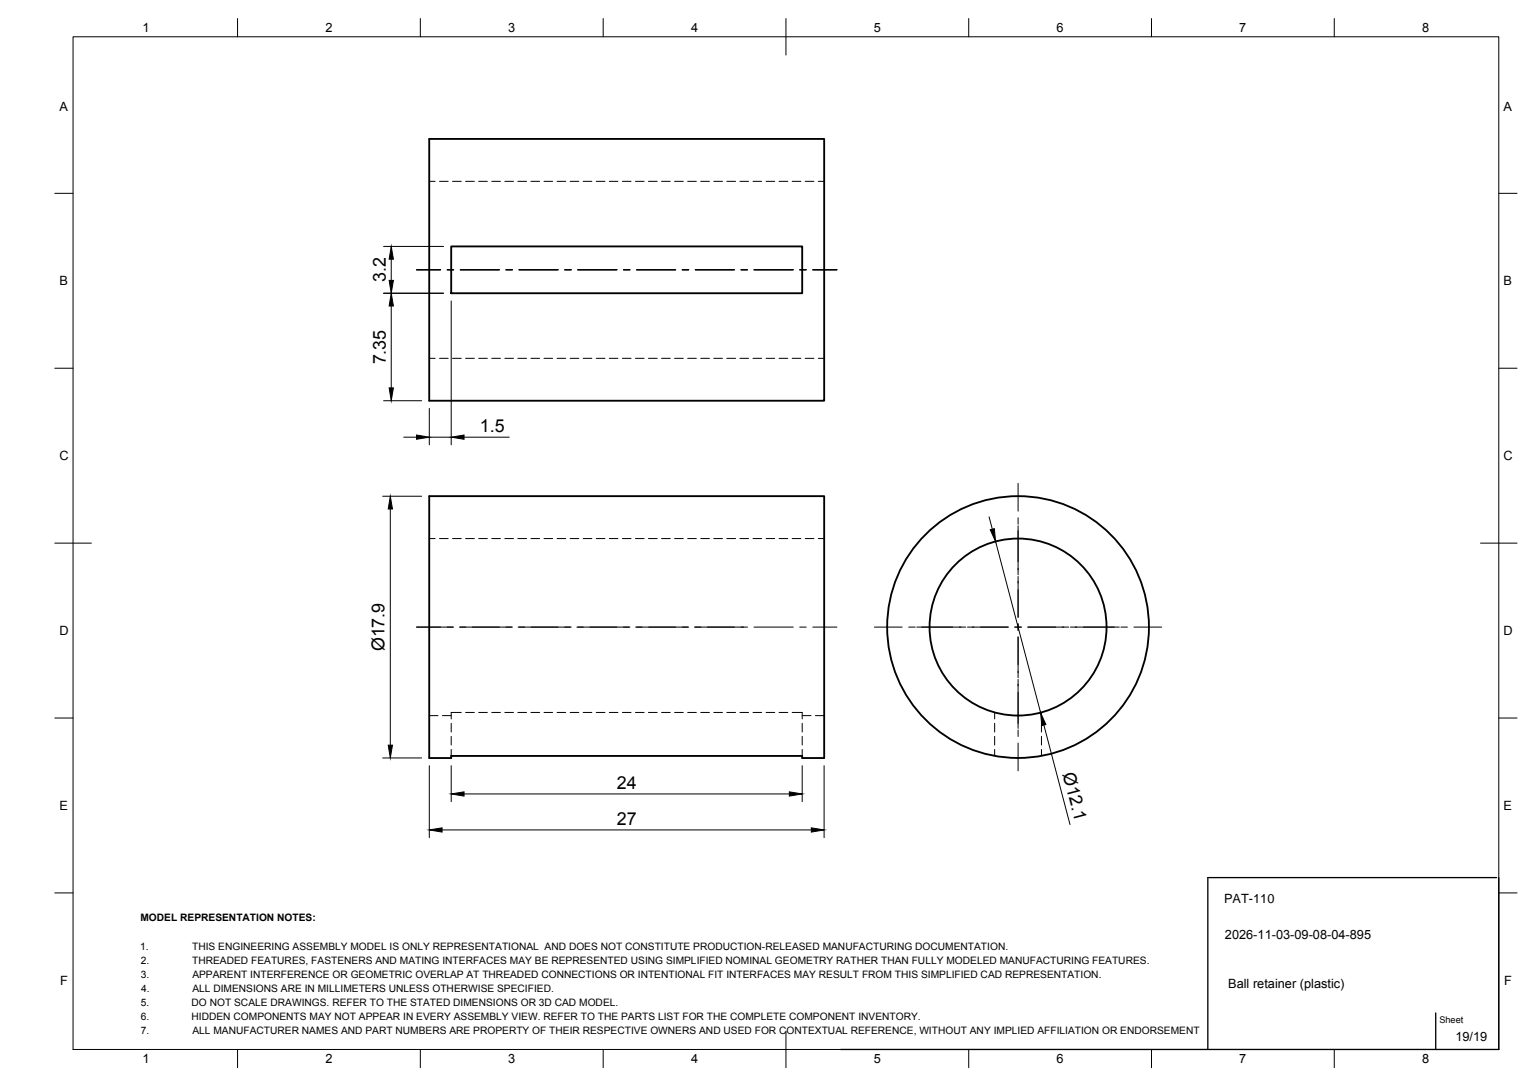
ISO-10303-21;
HEADER;
/* Generated by software containing ST-Developer
 * from STEP Tools, Inc. (www.steptools.com) 
 */

FILE_DESCRIPTION(
/* description */ ('Twin-shaft manual slide'),
/* implementation_level */ '2;1');

FILE_NAME(
/* name */ 'Ball retainer (plastic).step',
/* time_stamp */ '2026-10-27T18:38:08-07:00',
/* author */ (''),
/* organization */ (''),
/* preprocessor_version */ 'ST-DEVELOPER v20.2',
/* originating_system */ 'Autodesk Translation Framework v15.17.0.0',
/* authorisation */ '');

FILE_SCHEMA (('AUTOMOTIVE_DESIGN { 1 0 10303 214 3 1 1 }'));
ENDSEC;

DATA;
#10=MECHANICAL_DESIGN_GEOMETRIC_PRESENTATION_REPRESENTATION('',(#285),#6463);
#253=SHAPE_REPRESENTATION_RELATIONSHIP('SRR','None',#6573,#269);
#269=ADVANCED_BREP_SHAPE_REPRESENTATION('',(#300),#6456);
#285=STYLED_ITEM('',(#6733),#300);
#300=MANIFOLD_SOLID_BREP('Body1',#3648);
#378=FACE_BOUND('',#940,.T.);
#379=FACE_BOUND('',#942,.T.);
#380=FACE_BOUND('',#944,.T.);
#381=FACE_BOUND('',#946,.T.);
#477=PLANE('',#4078);
#478=PLANE('',#4081);
#479=PLANE('',#4082);
#480=PLANE('',#4085);
#481=PLANE('',#4086);
#482=PLANE('',#4091);
#654=FACE_OUTER_BOUND('',#935,.T.);
#655=FACE_OUTER_BOUND('',#936,.T.);
#656=FACE_OUTER_BOUND('',#937,.T.);
#657=FACE_OUTER_BOUND('',#938,.T.);
#658=FACE_OUTER_BOUND('',#939,.T.);
#659=FACE_OUTER_BOUND('',#941,.T.);
#660=FACE_OUTER_BOUND('',#943,.T.);
#661=FACE_OUTER_BOUND('',#945,.T.);
#935=EDGE_LOOP('',(#3054,#3055,#3056,#3057));
#936=EDGE_LOOP('',(#3058,#3059,#3060,#3061));
#937=EDGE_LOOP('',(#3062,#3063,#3064,#3065));
#938=EDGE_LOOP('',(#3066,#3067,#3068,#3069));
#939=EDGE_LOOP('',(#3070));
#940=EDGE_LOOP('',(#3071));
#941=EDGE_LOOP('',(#3072,#3073,#3074,#3075));
#942=EDGE_LOOP('',(#3076,#3077,#3078,#3079));
#943=EDGE_LOOP('',(#3080));
#944=EDGE_LOOP('',(#3081));
#945=EDGE_LOOP('',(#3082,#3083,#3084,#3085));
#946=EDGE_LOOP('',(#3086,#3087,#3088,#3089));
#1219=LINE('',#6034,#1505);
#1220=LINE('',#6037,#1506);
#1221=LINE('',#6040,#1507);
#1222=LINE('',#6042,#1508);
#1223=LINE('',#6043,#1509);
#1224=LINE('',#6049,#1510);
#1225=LINE('',#6051,#1511);
#1226=LINE('',#6052,#1512);
#1227=LINE('',#6061,#1513);
#1228=LINE('',#6066,#1514);
#1505=VECTOR('',#4939,1.);
#1506=VECTOR('',#4942,1.);
#1507=VECTOR('',#4945,1.);
#1508=VECTOR('',#4946,1.);
#1509=VECTOR('',#4947,1.);
#1510=VECTOR('',#4954,1.);
#1511=VECTOR('',#4957,1.);
#1512=VECTOR('',#4958,1.);
#1513=VECTOR('',#4969,0.895);
#1514=VECTOR('',#4976,0.605);
#1710=CIRCLE('',#4079,0.895);
#1711=CIRCLE('',#4080,0.605);
#1712=CIRCLE('',#4083,0.895);
#1713=CIRCLE('',#4084,0.605);
#1714=CIRCLE('',#4087,0.895);
#1715=CIRCLE('',#4088,0.605);
#1716=CIRCLE('',#4090,0.895);
#1717=CIRCLE('',#4092,0.605);
#1949=VERTEX_POINT('',#6030);
#1950=VERTEX_POINT('',#6031);
#1951=VERTEX_POINT('',#6033);
#1952=VERTEX_POINT('',#6035);
#1953=VERTEX_POINT('',#6039);
#1954=VERTEX_POINT('',#6041);
#1955=VERTEX_POINT('',#6045);
#1956=VERTEX_POINT('',#6047);
#1957=VERTEX_POINT('',#6054);
#1958=VERTEX_POINT('',#6056);
#1959=VERTEX_POINT('',#6059);
#1960=VERTEX_POINT('',#6063);
#2332=EDGE_CURVE('',#1949,#1950,#1710,.T.);
#2333=EDGE_CURVE('',#1951,#1949,#1219,.T.);
#2334=EDGE_CURVE('',#1952,#1951,#1711,.T.);
#2335=EDGE_CURVE('',#1950,#1952,#1220,.T.);
#2336=EDGE_CURVE('',#1950,#1953,#1221,.T.);
#2337=EDGE_CURVE('',#1954,#1952,#1222,.T.);
#2338=EDGE_CURVE('',#1954,#1953,#1223,.T.);
#2339=EDGE_CURVE('',#1953,#1955,#1712,.T.);
#2340=EDGE_CURVE('',#1956,#1954,#1713,.T.);
#2341=EDGE_CURVE('',#1955,#1956,#1224,.T.);
#2342=EDGE_CURVE('',#1955,#1949,#1225,.T.);
#2343=EDGE_CURVE('',#1951,#1956,#1226,.T.);
#2344=EDGE_CURVE('',#1957,#1957,#1714,.T.);
#2345=EDGE_CURVE('',#1958,#1958,#1715,.T.);
#2346=EDGE_CURVE('',#1959,#1959,#1716,.T.);
#2347=EDGE_CURVE('',#1959,#1957,#1227,.T.);
#2348=EDGE_CURVE('',#1960,#1960,#1717,.T.);
#2349=EDGE_CURVE('',#1960,#1958,#1228,.T.);
#3054=ORIENTED_EDGE('',*,*,#2332,.F.);
#3055=ORIENTED_EDGE('',*,*,#2333,.F.);
#3056=ORIENTED_EDGE('',*,*,#2334,.F.);
#3057=ORIENTED_EDGE('',*,*,#2335,.F.);
#3058=ORIENTED_EDGE('',*,*,#2336,.F.);
#3059=ORIENTED_EDGE('',*,*,#2335,.T.);
#3060=ORIENTED_EDGE('',*,*,#2337,.F.);
#3061=ORIENTED_EDGE('',*,*,#2338,.T.);
#3062=ORIENTED_EDGE('',*,*,#2339,.F.);
#3063=ORIENTED_EDGE('',*,*,#2338,.F.);
#3064=ORIENTED_EDGE('',*,*,#2340,.F.);
#3065=ORIENTED_EDGE('',*,*,#2341,.F.);
#3066=ORIENTED_EDGE('',*,*,#2342,.F.);
#3067=ORIENTED_EDGE('',*,*,#2341,.T.);
#3068=ORIENTED_EDGE('',*,*,#2343,.F.);
#3069=ORIENTED_EDGE('',*,*,#2333,.T.);
#3070=ORIENTED_EDGE('',*,*,#2344,.F.);
#3071=ORIENTED_EDGE('',*,*,#2345,.T.);
#3072=ORIENTED_EDGE('',*,*,#2346,.F.);
#3073=ORIENTED_EDGE('',*,*,#2347,.T.);
#3074=ORIENTED_EDGE('',*,*,#2344,.T.);
#3075=ORIENTED_EDGE('',*,*,#2347,.F.);
#3076=ORIENTED_EDGE('',*,*,#2339,.T.);
#3077=ORIENTED_EDGE('',*,*,#2342,.T.);
#3078=ORIENTED_EDGE('',*,*,#2332,.T.);
#3079=ORIENTED_EDGE('',*,*,#2336,.T.);
#3080=ORIENTED_EDGE('',*,*,#2346,.T.);
#3081=ORIENTED_EDGE('',*,*,#2348,.F.);
#3082=ORIENTED_EDGE('',*,*,#2348,.T.);
#3083=ORIENTED_EDGE('',*,*,#2349,.T.);
#3084=ORIENTED_EDGE('',*,*,#2345,.F.);
#3085=ORIENTED_EDGE('',*,*,#2349,.F.);
#3086=ORIENTED_EDGE('',*,*,#2340,.T.);
#3087=ORIENTED_EDGE('',*,*,#2337,.T.);
#3088=ORIENTED_EDGE('',*,*,#2334,.T.);
#3089=ORIENTED_EDGE('',*,*,#2343,.T.);
#3413=CYLINDRICAL_SURFACE('',#4089,0.895);
#3414=CYLINDRICAL_SURFACE('',#4093,0.605);
#3559=ADVANCED_FACE('',(#654),#477,.F.);
#3560=ADVANCED_FACE('',(#655),#478,.F.);
#3561=ADVANCED_FACE('',(#656),#479,.F.);
#3562=ADVANCED_FACE('',(#657),#480,.F.);
#3563=ADVANCED_FACE('',(#658,#378),#481,.T.);
#3564=ADVANCED_FACE('',(#659,#379),#3413,.T.);
#3565=ADVANCED_FACE('',(#660,#380),#482,.T.);
#3566=ADVANCED_FACE('',(#661,#381),#3414,.F.);
#3648=CLOSED_SHELL('',(#3559,#3560,#3561,#3562,#3563,#3564,#3565,#3566));
#4077=AXIS2_PLACEMENT_3D('',#6028,#4933,#4934);
#4078=AXIS2_PLACEMENT_3D('',#6029,#4935,#4936);
#4079=AXIS2_PLACEMENT_3D('',#6032,#4937,#4938);
#4080=AXIS2_PLACEMENT_3D('',#6036,#4940,#4941);
#4081=AXIS2_PLACEMENT_3D('',#6038,#4943,#4944);
#4082=AXIS2_PLACEMENT_3D('',#6044,#4948,#4949);
#4083=AXIS2_PLACEMENT_3D('',#6046,#4950,#4951);
#4084=AXIS2_PLACEMENT_3D('',#6048,#4952,#4953);
#4085=AXIS2_PLACEMENT_3D('',#6050,#4955,#4956);
#4086=AXIS2_PLACEMENT_3D('',#6053,#4959,#4960);
#4087=AXIS2_PLACEMENT_3D('',#6055,#4961,#4962);
#4088=AXIS2_PLACEMENT_3D('',#6057,#4963,#4964);
#4089=AXIS2_PLACEMENT_3D('',#6058,#4965,#4966);
#4090=AXIS2_PLACEMENT_3D('',#6060,#4967,#4968);
#4091=AXIS2_PLACEMENT_3D('',#6062,#4970,#4971);
#4092=AXIS2_PLACEMENT_3D('',#6064,#4972,#4973);
#4093=AXIS2_PLACEMENT_3D('',#6065,#4974,#4975);
#4933=DIRECTION('axis',(0.,0.,1.));
#4934=DIRECTION('refdir',(1.,0.,0.));
#4935=DIRECTION('center_axis',(0.,1.,0.));
#4936=DIRECTION('ref_axis',(0.,0.,1.));
#4937=DIRECTION('center_axis',(0.,1.,0.));
#4938=DIRECTION('ref_axis',(1.,0.,0.));
#4939=DIRECTION('',(1.,0.,0.));
#4940=DIRECTION('center_axis',(0.,-1.,0.));
#4941=DIRECTION('ref_axis',(1.,0.,0.));
#4942=DIRECTION('',(-1.,0.,0.));
#4943=DIRECTION('center_axis',(0.,0.,-1.));
#4944=DIRECTION('ref_axis',(-1.,0.,0.));
#4945=DIRECTION('',(0.,-1.,0.));
#4946=DIRECTION('',(0.,1.,0.));
#4947=DIRECTION('',(1.,0.,0.));
#4948=DIRECTION('center_axis',(0.,-1.,0.));
#4949=DIRECTION('ref_axis',(0.,0.,-1.));
#4950=DIRECTION('center_axis',(0.,-1.,0.));
#4951=DIRECTION('ref_axis',(1.,0.,0.));
#4952=DIRECTION('center_axis',(0.,1.,0.));
#4953=DIRECTION('ref_axis',(1.,0.,0.));
#4954=DIRECTION('',(-1.,0.,0.));
#4955=DIRECTION('center_axis',(0.,0.,1.));
#4956=DIRECTION('ref_axis',(1.,0.,0.));
#4957=DIRECTION('',(0.,1.,0.));
#4958=DIRECTION('',(0.,-1.,0.));
#4959=DIRECTION('center_axis',(0.,1.,0.));
#4960=DIRECTION('ref_axis',(0.,0.,1.));
#4961=DIRECTION('center_axis',(0.,-1.,0.));
#4962=DIRECTION('ref_axis',(1.,0.,0.));
#4963=DIRECTION('center_axis',(0.,-1.,0.));
#4964=DIRECTION('ref_axis',(1.,0.,0.));
#4965=DIRECTION('center_axis',(0.,-1.,0.));
#4966=DIRECTION('ref_axis',(1.,0.,0.));
#4967=DIRECTION('center_axis',(0.,-1.,0.));
#4968=DIRECTION('ref_axis',(1.,0.,0.));
#4969=DIRECTION('',(0.,1.,0.));
#4970=DIRECTION('center_axis',(0.,-1.,0.));
#4971=DIRECTION('ref_axis',(0.,0.,-1.));
#4972=DIRECTION('center_axis',(0.,-1.,0.));
#4973=DIRECTION('ref_axis',(1.,0.,0.));
#4974=DIRECTION('center_axis',(0.,-1.,0.));
#4975=DIRECTION('ref_axis',(1.,0.,0.));
#4976=DIRECTION('',(0.,1.,0.));
#6028=CARTESIAN_POINT('',(0.,0.,0.));
#6029=CARTESIAN_POINT('Origin',(0.75,1.2,0.));
#6030=CARTESIAN_POINT('',(0.880582193778639,1.2,0.16));
#6031=CARTESIAN_POINT('',(0.880582193778639,1.2,-0.16));
#6032=CARTESIAN_POINT('Origin',(0.,1.2,0.));
#6033=CARTESIAN_POINT('',(0.583459510163302,1.2,0.16));
#6034=CARTESIAN_POINT('',(0.57,1.2,0.16));
#6035=CARTESIAN_POINT('',(0.583459510163302,1.2,-0.16));
#6036=CARTESIAN_POINT('Origin',(0.,1.2,0.));
#6037=CARTESIAN_POINT('',(0.93,1.2,-0.16));
#6038=CARTESIAN_POINT('Origin',(0.93,0.,-0.16));
#6039=CARTESIAN_POINT('',(0.880582193778639,-1.2,-0.16));
#6040=CARTESIAN_POINT('',(0.880582193778639,0.,-0.16));
#6041=CARTESIAN_POINT('',(0.583459510163302,-1.2,-0.16));
#6042=CARTESIAN_POINT('',(0.583459510163302,0.,-0.16));
#6043=CARTESIAN_POINT('',(0.93,-1.2,-0.16));
#6044=CARTESIAN_POINT('Origin',(0.75,-1.2,0.));
#6045=CARTESIAN_POINT('',(0.880582193778639,-1.2,0.16));
#6046=CARTESIAN_POINT('Origin',(0.,-1.2,0.));
#6047=CARTESIAN_POINT('',(0.583459510163302,-1.2,0.16));
#6048=CARTESIAN_POINT('Origin',(0.,-1.2,0.));
#6049=CARTESIAN_POINT('',(0.57,-1.2,0.16));
#6050=CARTESIAN_POINT('Origin',(0.57,0.,0.16));
#6051=CARTESIAN_POINT('',(0.880582193778639,0.,0.16));
#6052=CARTESIAN_POINT('',(0.583459510163302,0.,0.16));
#6053=CARTESIAN_POINT('Origin',(0.895,1.35,0.));
#6054=CARTESIAN_POINT('',(-0.895,1.35,-1.09605888523688E-16));
#6055=CARTESIAN_POINT('Origin',(0.,1.35,0.));
#6056=CARTESIAN_POINT('',(-0.605,1.35,-7.40911313484149E-17));
#6057=CARTESIAN_POINT('Origin',(0.,1.35,0.));
#6058=CARTESIAN_POINT('Origin',(0.,0.,0.));
#6059=CARTESIAN_POINT('',(-0.895,-1.35,-1.09605888523688E-16));
#6060=CARTESIAN_POINT('Origin',(0.,-1.35,0.));
#6061=CARTESIAN_POINT('',(-0.895,0.,-1.09605888523688E-16));
#6062=CARTESIAN_POINT('Origin',(0.605,-1.35,0.));
#6063=CARTESIAN_POINT('',(-0.605,-1.35,-7.40911313484149E-17));
#6064=CARTESIAN_POINT('Origin',(0.,-1.35,0.));
#6065=CARTESIAN_POINT('Origin',(0.,0.,0.));
#6066=CARTESIAN_POINT('',(-0.605,0.,-7.40911313484149E-17));
#6435=UNCERTAINTY_MEASURE_WITH_UNIT(LENGTH_MEASURE(0.001),#6464,
'DISTANCE_ACCURACY_VALUE',
'Maximum model space distance between geometric entities at asserted c
onnectivities');
#6442=UNCERTAINTY_MEASURE_WITH_UNIT(LENGTH_MEASURE(0.001),#6464,
'DISTANCE_ACCURACY_VALUE',
'Maximum model space distance between geometric entities at asserted c
onnectivities');
#6456=(
GEOMETRIC_REPRESENTATION_CONTEXT(3)
GLOBAL_UNCERTAINTY_ASSIGNED_CONTEXT((#6435))
GLOBAL_UNIT_ASSIGNED_CONTEXT((#6464,#6466,#6467))
REPRESENTATION_CONTEXT('','3D')
);
#6463=(
GEOMETRIC_REPRESENTATION_CONTEXT(3)
GLOBAL_UNCERTAINTY_ASSIGNED_CONTEXT((#6442))
GLOBAL_UNIT_ASSIGNED_CONTEXT((#6464,#6466,#6467))
REPRESENTATION_CONTEXT('','3D')
);
#6464=(
LENGTH_UNIT()
NAMED_UNIT(*)
SI_UNIT(.CENTI.,.METRE.)
);
#6466=(
NAMED_UNIT(*)
PLANE_ANGLE_UNIT()
SI_UNIT($,.RADIAN.)
);
#6467=(
NAMED_UNIT(*)
SI_UNIT($,.STERADIAN.)
SOLID_ANGLE_UNIT()
);
#6481=SHAPE_DEFINITION_REPRESENTATION(#6501,#6573);
#6501=PRODUCT_DEFINITION_SHAPE('',$,#6594);
#6573=SHAPE_REPRESENTATION('',(#4077),#6456);
#6580=PRODUCT_DEFINITION_CONTEXT('part definition',#6642,'design');
#6594=PRODUCT_DEFINITION('Ball retainer (plastic)',
'Ball retainer (plastic)',#6614,#6580);
#6614=PRODUCT_DEFINITION_FORMATION('',$,#6657);
#6642=APPLICATION_CONTEXT(
'Core Data for Automotive Mechanical Design Process');
#6643=PRODUCT_CONTEXT('part definition',#6642,'mechanical');
#6657=PRODUCT('Ball retainer (plastic)','Ball retainer (plastic)',
'Ball retainer (plastic)',(#6643));
#6727=COLOUR_RGB('Sky Blue',0.24,0.69,0.87);
#6728=FILL_AREA_STYLE_COLOUR('',#6727);
#6729=FILL_AREA_STYLE('',(#6728));
#6730=SURFACE_STYLE_FILL_AREA(#6729);
#6731=SURFACE_SIDE_STYLE('',(#6730));
#6732=SURFACE_STYLE_USAGE(.BOTH.,#6731);
#6733=PRESENTATION_STYLE_ASSIGNMENT((#6732));
ENDSEC;
END-ISO-10303-21;
